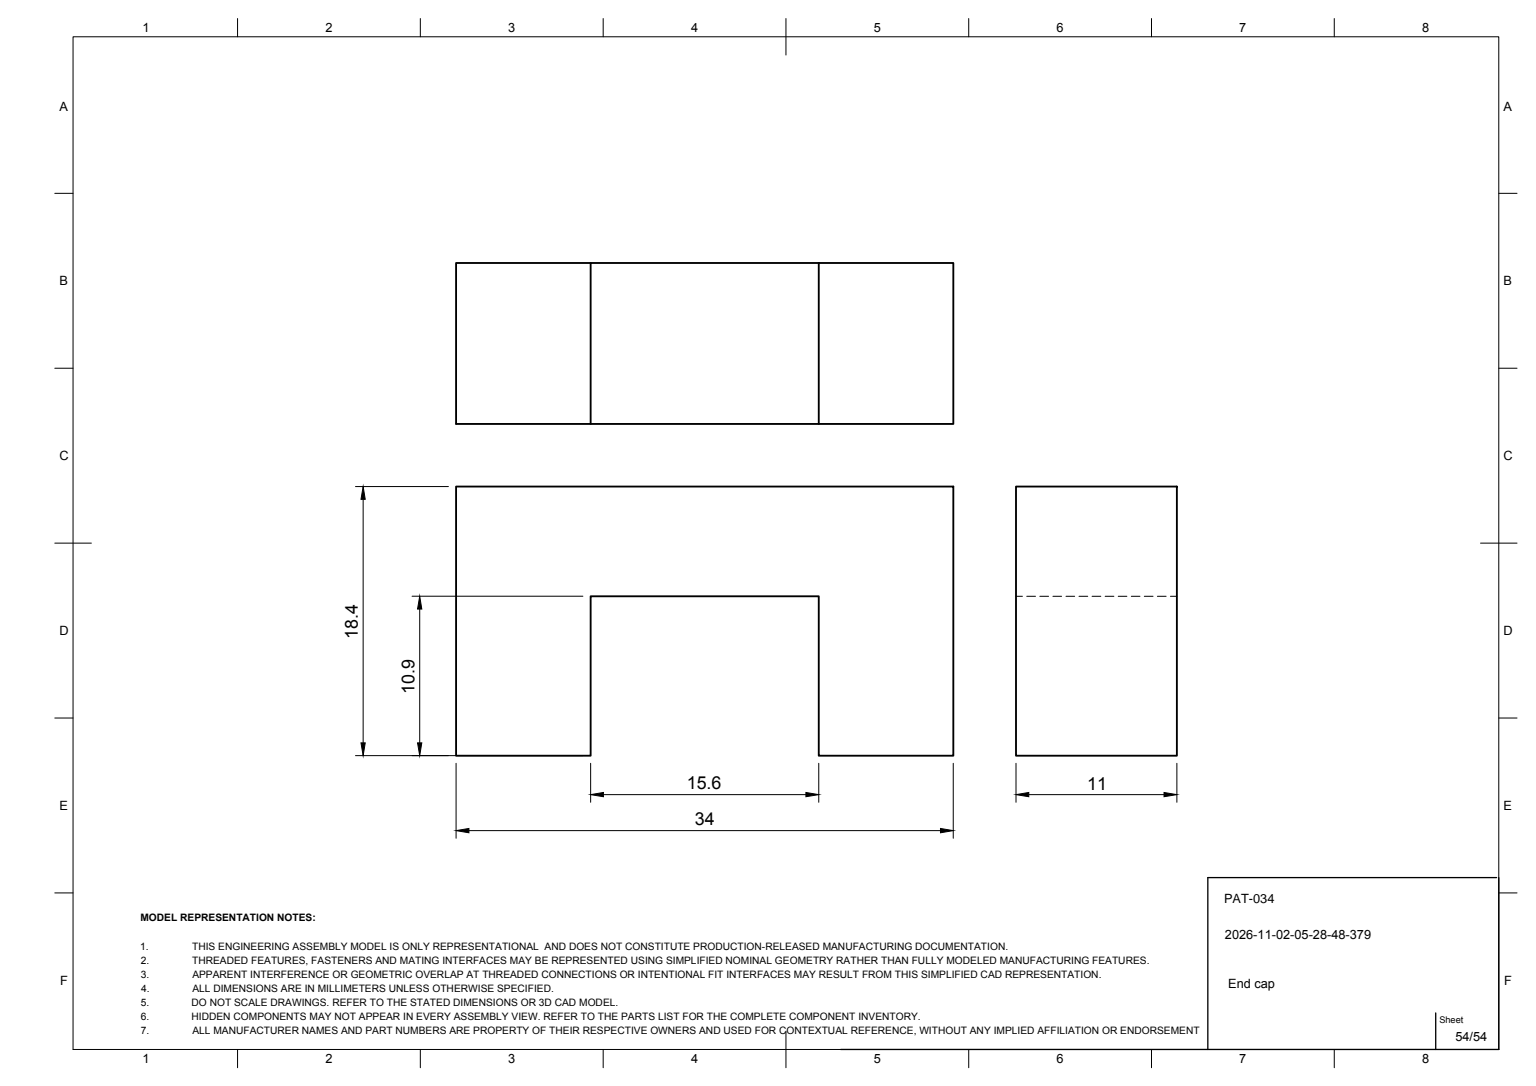
ISO-10303-21;
HEADER;
/* Generated by software containing ST-Developer
 * from STEP Tools, Inc. (www.steptools.com) 
 */

FILE_DESCRIPTION(
/* description */ ('Fatigue rig crank-slider'),
/* implementation_level */ '2;1');

FILE_NAME(
/* name */ 'End cap.step',
/* time_stamp */ '2026-10-28T03:24:50-07:00',
/* author */ (''),
/* organization */ (''),
/* preprocessor_version */ 'ST-DEVELOPER v20.2',
/* originating_system */ 'Autodesk Translation Framework v15.17.0.0',
/* authorisation */ '');

FILE_SCHEMA (('AUTOMOTIVE_DESIGN { 1 0 10303 214 3 1 1 }'));
ENDSEC;

DATA;
#10=MECHANICAL_DESIGN_GEOMETRIC_PRESENTATION_REPRESENTATION('',(#641),#16911);
#532=SHAPE_REPRESENTATION_RELATIONSHIP('SRR','None',#17177,#582);
#582=ADVANCED_BREP_SHAPE_REPRESENTATION('',(#698),#16906);
#641=STYLED_ITEM('',(#17501),#698);
#698=MANIFOLD_SOLID_BREP('Body1',#8934);
#1172=PLANE('',#10393);
#1173=PLANE('',#10394);
#1174=PLANE('',#10395);
#1175=PLANE('',#10396);
#1176=PLANE('',#10397);
#1177=PLANE('',#10398);
#1178=PLANE('',#10399);
#1179=PLANE('',#10400);
#1180=PLANE('',#10401);
#1181=PLANE('',#10402);
#1676=FACE_OUTER_BOUND('',#2391,.T.);
#1677=FACE_OUTER_BOUND('',#2392,.T.);
#1678=FACE_OUTER_BOUND('',#2393,.T.);
#1679=FACE_OUTER_BOUND('',#2394,.T.);
#1680=FACE_OUTER_BOUND('',#2395,.T.);
#1681=FACE_OUTER_BOUND('',#2396,.T.);
#1682=FACE_OUTER_BOUND('',#2397,.T.);
#1683=FACE_OUTER_BOUND('',#2398,.T.);
#1684=FACE_OUTER_BOUND('',#2399,.T.);
#1685=FACE_OUTER_BOUND('',#2400,.T.);
#2391=EDGE_LOOP('',(#7948,#7949,#7950,#7951));
#2392=EDGE_LOOP('',(#7952,#7953,#7954,#7955));
#2393=EDGE_LOOP('',(#7956,#7957,#7958,#7959));
#2394=EDGE_LOOP('',(#7960,#7961,#7962,#7963));
#2395=EDGE_LOOP('',(#7964,#7965,#7966,#7967));
#2396=EDGE_LOOP('',(#7968,#7969,#7970,#7971));
#2397=EDGE_LOOP('',(#7972,#7973,#7974,#7975));
#2398=EDGE_LOOP('',(#7976,#7977,#7978,#7979));
#2399=EDGE_LOOP('',(#7980,#7981,#7982,#7983,#7984,#7985,#7986,#7987));
#2400=EDGE_LOOP('',(#7988,#7989,#7990,#7991,#7992,#7993,#7994,#7995));
#3009=LINE('',#16448,#3655);
#3010=LINE('',#16450,#3656);
#3011=LINE('',#16452,#3657);
#3012=LINE('',#16453,#3658);
#3013=LINE('',#16456,#3659);
#3014=LINE('',#16458,#3660);
#3015=LINE('',#16459,#3661);
#3016=LINE('',#16462,#3662);
#3017=LINE('',#16464,#3663);
#3018=LINE('',#16465,#3664);
#3019=LINE('',#16468,#3665);
#3020=LINE('',#16470,#3666);
#3021=LINE('',#16471,#3667);
#3022=LINE('',#16474,#3668);
#3023=LINE('',#16476,#3669);
#3024=LINE('',#16477,#3670);
#3025=LINE('',#16480,#3671);
#3026=LINE('',#16482,#3672);
#3027=LINE('',#16483,#3673);
#3028=LINE('',#16486,#3674);
#3029=LINE('',#16488,#3675);
#3030=LINE('',#16489,#3676);
#3031=LINE('',#16491,#3677);
#3032=LINE('',#16492,#3678);
#3655=VECTOR('',#12917,1.);
#3656=VECTOR('',#12918,1.);
#3657=VECTOR('',#12919,1.);
#3658=VECTOR('',#12920,1.);
#3659=VECTOR('',#12923,1.);
#3660=VECTOR('',#12924,1.);
#3661=VECTOR('',#12925,1.);
#3662=VECTOR('',#12928,1.);
#3663=VECTOR('',#12929,1.);
#3664=VECTOR('',#12930,1.);
#3665=VECTOR('',#12933,1.);
#3666=VECTOR('',#12934,1.);
#3667=VECTOR('',#12935,1.);
#3668=VECTOR('',#12938,1.);
#3669=VECTOR('',#12939,1.);
#3670=VECTOR('',#12940,1.);
#3671=VECTOR('',#12943,1.);
#3672=VECTOR('',#12944,1.);
#3673=VECTOR('',#12945,1.);
#3674=VECTOR('',#12948,1.);
#3675=VECTOR('',#12949,1.);
#3676=VECTOR('',#12950,1.);
#3677=VECTOR('',#12953,1.);
#3678=VECTOR('',#12954,1.);
#4817=VERTEX_POINT('',#16446);
#4818=VERTEX_POINT('',#16447);
#4819=VERTEX_POINT('',#16449);
#4820=VERTEX_POINT('',#16451);
#4821=VERTEX_POINT('',#16455);
#4822=VERTEX_POINT('',#16457);
#4823=VERTEX_POINT('',#16461);
#4824=VERTEX_POINT('',#16463);
#4825=VERTEX_POINT('',#16467);
#4826=VERTEX_POINT('',#16469);
#4827=VERTEX_POINT('',#16473);
#4828=VERTEX_POINT('',#16475);
#4829=VERTEX_POINT('',#16479);
#4830=VERTEX_POINT('',#16481);
#4831=VERTEX_POINT('',#16485);
#4832=VERTEX_POINT('',#16487);
#5872=EDGE_CURVE('',#4817,#4818,#3009,.T.);
#5873=EDGE_CURVE('',#4817,#4819,#3010,.T.);
#5874=EDGE_CURVE('',#4820,#4819,#3011,.T.);
#5875=EDGE_CURVE('',#4818,#4820,#3012,.T.);
#5876=EDGE_CURVE('',#4818,#4821,#3013,.T.);
#5877=EDGE_CURVE('',#4822,#4820,#3014,.T.);
#5878=EDGE_CURVE('',#4821,#4822,#3015,.T.);
#5879=EDGE_CURVE('',#4821,#4823,#3016,.T.);
#5880=EDGE_CURVE('',#4824,#4822,#3017,.T.);
#5881=EDGE_CURVE('',#4823,#4824,#3018,.T.);
#5882=EDGE_CURVE('',#4823,#4825,#3019,.T.);
#5883=EDGE_CURVE('',#4826,#4824,#3020,.T.);
#5884=EDGE_CURVE('',#4825,#4826,#3021,.T.);
#5885=EDGE_CURVE('',#4825,#4827,#3022,.T.);
#5886=EDGE_CURVE('',#4828,#4826,#3023,.T.);
#5887=EDGE_CURVE('',#4827,#4828,#3024,.T.);
#5888=EDGE_CURVE('',#4827,#4829,#3025,.T.);
#5889=EDGE_CURVE('',#4830,#4828,#3026,.T.);
#5890=EDGE_CURVE('',#4829,#4830,#3027,.T.);
#5891=EDGE_CURVE('',#4829,#4831,#3028,.T.);
#5892=EDGE_CURVE('',#4832,#4830,#3029,.T.);
#5893=EDGE_CURVE('',#4831,#4832,#3030,.T.);
#5894=EDGE_CURVE('',#4831,#4817,#3031,.T.);
#5895=EDGE_CURVE('',#4819,#4832,#3032,.T.);
#7948=ORIENTED_EDGE('',*,*,#5872,.F.);
#7949=ORIENTED_EDGE('',*,*,#5873,.T.);
#7950=ORIENTED_EDGE('',*,*,#5874,.F.);
#7951=ORIENTED_EDGE('',*,*,#5875,.F.);
#7952=ORIENTED_EDGE('',*,*,#5876,.F.);
#7953=ORIENTED_EDGE('',*,*,#5875,.T.);
#7954=ORIENTED_EDGE('',*,*,#5877,.F.);
#7955=ORIENTED_EDGE('',*,*,#5878,.F.);
#7956=ORIENTED_EDGE('',*,*,#5879,.F.);
#7957=ORIENTED_EDGE('',*,*,#5878,.T.);
#7958=ORIENTED_EDGE('',*,*,#5880,.F.);
#7959=ORIENTED_EDGE('',*,*,#5881,.F.);
#7960=ORIENTED_EDGE('',*,*,#5882,.F.);
#7961=ORIENTED_EDGE('',*,*,#5881,.T.);
#7962=ORIENTED_EDGE('',*,*,#5883,.F.);
#7963=ORIENTED_EDGE('',*,*,#5884,.F.);
#7964=ORIENTED_EDGE('',*,*,#5885,.F.);
#7965=ORIENTED_EDGE('',*,*,#5884,.T.);
#7966=ORIENTED_EDGE('',*,*,#5886,.F.);
#7967=ORIENTED_EDGE('',*,*,#5887,.F.);
#7968=ORIENTED_EDGE('',*,*,#5888,.F.);
#7969=ORIENTED_EDGE('',*,*,#5887,.T.);
#7970=ORIENTED_EDGE('',*,*,#5889,.F.);
#7971=ORIENTED_EDGE('',*,*,#5890,.F.);
#7972=ORIENTED_EDGE('',*,*,#5891,.F.);
#7973=ORIENTED_EDGE('',*,*,#5890,.T.);
#7974=ORIENTED_EDGE('',*,*,#5892,.F.);
#7975=ORIENTED_EDGE('',*,*,#5893,.F.);
#7976=ORIENTED_EDGE('',*,*,#5894,.F.);
#7977=ORIENTED_EDGE('',*,*,#5893,.T.);
#7978=ORIENTED_EDGE('',*,*,#5895,.F.);
#7979=ORIENTED_EDGE('',*,*,#5873,.F.);
#7980=ORIENTED_EDGE('',*,*,#5894,.T.);
#7981=ORIENTED_EDGE('',*,*,#5872,.T.);
#7982=ORIENTED_EDGE('',*,*,#5876,.T.);
#7983=ORIENTED_EDGE('',*,*,#5879,.T.);
#7984=ORIENTED_EDGE('',*,*,#5882,.T.);
#7985=ORIENTED_EDGE('',*,*,#5885,.T.);
#7986=ORIENTED_EDGE('',*,*,#5888,.T.);
#7987=ORIENTED_EDGE('',*,*,#5891,.T.);
#7988=ORIENTED_EDGE('',*,*,#5895,.T.);
#7989=ORIENTED_EDGE('',*,*,#5892,.T.);
#7990=ORIENTED_EDGE('',*,*,#5889,.T.);
#7991=ORIENTED_EDGE('',*,*,#5886,.T.);
#7992=ORIENTED_EDGE('',*,*,#5883,.T.);
#7993=ORIENTED_EDGE('',*,*,#5880,.T.);
#7994=ORIENTED_EDGE('',*,*,#5877,.T.);
#7995=ORIENTED_EDGE('',*,*,#5874,.T.);
#8814=ADVANCED_FACE('',(#1676),#1172,.T.);
#8815=ADVANCED_FACE('',(#1677),#1173,.T.);
#8816=ADVANCED_FACE('',(#1678),#1174,.T.);
#8817=ADVANCED_FACE('',(#1679),#1175,.T.);
#8818=ADVANCED_FACE('',(#1680),#1176,.T.);
#8819=ADVANCED_FACE('',(#1681),#1177,.T.);
#8820=ADVANCED_FACE('',(#1682),#1178,.T.);
#8821=ADVANCED_FACE('',(#1683),#1179,.T.);
#8822=ADVANCED_FACE('',(#1684),#1180,.T.);
#8823=ADVANCED_FACE('',(#1685),#1181,.T.);
#8934=CLOSED_SHELL('',(#8814,#8815,#8816,#8817,#8818,#8819,#8820,#8821,
#8822,#8823));
#10392=AXIS2_PLACEMENT_3D('',#16444,#12913,#12914);
#10393=AXIS2_PLACEMENT_3D('',#16445,#12915,#12916);
#10394=AXIS2_PLACEMENT_3D('',#16454,#12921,#12922);
#10395=AXIS2_PLACEMENT_3D('',#16460,#12926,#12927);
#10396=AXIS2_PLACEMENT_3D('',#16466,#12931,#12932);
#10397=AXIS2_PLACEMENT_3D('',#16472,#12936,#12937);
#10398=AXIS2_PLACEMENT_3D('',#16478,#12941,#12942);
#10399=AXIS2_PLACEMENT_3D('',#16484,#12946,#12947);
#10400=AXIS2_PLACEMENT_3D('',#16490,#12951,#12952);
#10401=AXIS2_PLACEMENT_3D('',#16493,#12955,#12956);
#10402=AXIS2_PLACEMENT_3D('',#16494,#12957,#12958);
#12913=DIRECTION('axis',(0.,0.,1.));
#12914=DIRECTION('refdir',(1.,0.,0.));
#12915=DIRECTION('center_axis',(0.,0.,-1.));
#12916=DIRECTION('ref_axis',(0.,-1.,0.));
#12917=DIRECTION('',(0.,1.,0.));
#12918=DIRECTION('',(-1.,0.,0.));
#12919=DIRECTION('',(0.,-1.,0.));
#12920=DIRECTION('',(-1.,0.,0.));
#12921=DIRECTION('center_axis',(0.,1.,0.));
#12922=DIRECTION('ref_axis',(0.,0.,-1.));
#12923=DIRECTION('',(0.,0.,1.));
#12924=DIRECTION('',(0.,0.,-1.));
#12925=DIRECTION('',(-1.,0.,0.));
#12926=DIRECTION('center_axis',(0.,0.,-1.));
#12927=DIRECTION('ref_axis',(0.,-1.,0.));
#12928=DIRECTION('',(0.,1.,0.));
#12929=DIRECTION('',(0.,-1.,0.));
#12930=DIRECTION('',(-1.,0.,0.));
#12931=DIRECTION('center_axis',(0.,-1.,0.));
#12932=DIRECTION('ref_axis',(0.,0.,1.));
#12933=DIRECTION('',(0.,0.,-1.));
#12934=DIRECTION('',(0.,0.,1.));
#12935=DIRECTION('',(-1.,0.,0.));
#12936=DIRECTION('center_axis',(0.,0.,-1.));
#12937=DIRECTION('ref_axis',(0.,-1.,0.));
#12938=DIRECTION('',(0.,1.,0.));
#12939=DIRECTION('',(0.,-1.,0.));
#12940=DIRECTION('',(-1.,0.,0.));
#12941=DIRECTION('center_axis',(0.,1.,0.));
#12942=DIRECTION('ref_axis',(0.,0.,-1.));
#12943=DIRECTION('',(0.,0.,1.));
#12944=DIRECTION('',(0.,0.,-1.));
#12945=DIRECTION('',(-1.,0.,0.));
#12946=DIRECTION('center_axis',(0.,0.,1.));
#12947=DIRECTION('ref_axis',(0.,1.,0.));
#12948=DIRECTION('',(0.,-1.,0.));
#12949=DIRECTION('',(0.,1.,0.));
#12950=DIRECTION('',(-1.,0.,0.));
#12951=DIRECTION('center_axis',(0.,-1.,0.));
#12952=DIRECTION('ref_axis',(0.,0.,1.));
#12953=DIRECTION('',(0.,0.,-1.));
#12954=DIRECTION('',(0.,0.,1.));
#12955=DIRECTION('center_axis',(1.,0.,0.));
#12956=DIRECTION('ref_axis',(0.,0.,-1.));
#12957=DIRECTION('center_axis',(-1.,0.,0.));
#12958=DIRECTION('ref_axis',(0.,0.,1.));
#16444=CARTESIAN_POINT('',(0.,0.,0.));
#16445=CARTESIAN_POINT('Origin',(-1.97,-0.78,0.46));
#16446=CARTESIAN_POINT('',(-1.97,-1.7,0.46));
#16447=CARTESIAN_POINT('',(-1.97,-0.78,0.46));
#16448=CARTESIAN_POINT('',(-1.97,-1.7,0.46));
#16449=CARTESIAN_POINT('',(-3.07,-1.7,0.46));
#16450=CARTESIAN_POINT('',(-1.97,-1.7,0.46));
#16451=CARTESIAN_POINT('',(-3.07,-0.78,0.46));
#16452=CARTESIAN_POINT('',(-3.07,-1.7,0.46));
#16453=CARTESIAN_POINT('',(-1.97,-0.78,0.46));
#16454=CARTESIAN_POINT('Origin',(-1.97,-0.78,1.55));
#16455=CARTESIAN_POINT('',(-1.97,-0.78,1.55));
#16456=CARTESIAN_POINT('',(-1.97,-0.78,0.46));
#16457=CARTESIAN_POINT('',(-3.07,-0.78,1.55));
#16458=CARTESIAN_POINT('',(-3.07,-0.78,0.46));
#16459=CARTESIAN_POINT('',(-1.97,-0.78,1.55));
#16460=CARTESIAN_POINT('Origin',(-1.97,0.78,1.55));
#16461=CARTESIAN_POINT('',(-1.97,0.78,1.55));
#16462=CARTESIAN_POINT('',(-1.97,-0.78,1.55));
#16463=CARTESIAN_POINT('',(-3.07,0.78,1.55));
#16464=CARTESIAN_POINT('',(-3.07,-0.78,1.55));
#16465=CARTESIAN_POINT('',(-1.97,0.78,1.55));
#16466=CARTESIAN_POINT('Origin',(-1.97,0.78,0.46));
#16467=CARTESIAN_POINT('',(-1.97,0.78,0.46));
#16468=CARTESIAN_POINT('',(-1.97,0.78,1.55));
#16469=CARTESIAN_POINT('',(-3.07,0.78,0.46));
#16470=CARTESIAN_POINT('',(-3.07,0.78,1.55));
#16471=CARTESIAN_POINT('',(-1.97,0.78,0.46));
#16472=CARTESIAN_POINT('Origin',(-1.97,1.7,0.46));
#16473=CARTESIAN_POINT('',(-1.97,1.7,0.46));
#16474=CARTESIAN_POINT('',(-1.97,0.78,0.46));
#16475=CARTESIAN_POINT('',(-3.07,1.7,0.46));
#16476=CARTESIAN_POINT('',(-3.07,0.78,0.46));
#16477=CARTESIAN_POINT('',(-1.97,1.7,0.46));
#16478=CARTESIAN_POINT('Origin',(-1.97,1.7,2.3));
#16479=CARTESIAN_POINT('',(-1.97,1.7,2.3));
#16480=CARTESIAN_POINT('',(-1.97,1.7,0.46));
#16481=CARTESIAN_POINT('',(-3.07,1.7,2.3));
#16482=CARTESIAN_POINT('',(-3.07,1.7,0.46));
#16483=CARTESIAN_POINT('',(-1.97,1.7,2.3));
#16484=CARTESIAN_POINT('Origin',(-1.97,-1.7,2.3));
#16485=CARTESIAN_POINT('',(-1.97,-1.7,2.3));
#16486=CARTESIAN_POINT('',(-1.97,1.7,2.3));
#16487=CARTESIAN_POINT('',(-3.07,-1.7,2.3));
#16488=CARTESIAN_POINT('',(-3.07,1.7,2.3));
#16489=CARTESIAN_POINT('',(-1.97,-1.7,2.3));
#16490=CARTESIAN_POINT('Origin',(-1.97,-1.7,0.46));
#16491=CARTESIAN_POINT('',(-1.97,-1.7,2.3));
#16492=CARTESIAN_POINT('',(-3.07,-1.7,2.3));
#16493=CARTESIAN_POINT('Origin',(-1.97,0.,1.38));
#16494=CARTESIAN_POINT('Origin',(-3.07,0.,1.38));
#16847=UNCERTAINTY_MEASURE_WITH_UNIT(LENGTH_MEASURE(0.001),#16912,
'DISTANCE_ACCURACY_VALUE',
'Maximum model space distance between geometric entities at asserted c
onnectivities');
#16852=UNCERTAINTY_MEASURE_WITH_UNIT(LENGTH_MEASURE(0.001),#16912,
'DISTANCE_ACCURACY_VALUE',
'Maximum model space distance between geometric entities at asserted c
onnectivities');
#16906=(
GEOMETRIC_REPRESENTATION_CONTEXT(3)
GLOBAL_UNCERTAINTY_ASSIGNED_CONTEXT((#16847))
GLOBAL_UNIT_ASSIGNED_CONTEXT((#16912,#16914,#16915))
REPRESENTATION_CONTEXT('','3D')
);
#16911=(
GEOMETRIC_REPRESENTATION_CONTEXT(3)
GLOBAL_UNCERTAINTY_ASSIGNED_CONTEXT((#16852))
GLOBAL_UNIT_ASSIGNED_CONTEXT((#16912,#16914,#16915))
REPRESENTATION_CONTEXT('','3D')
);
#16912=(
LENGTH_UNIT()
NAMED_UNIT(*)
SI_UNIT(.CENTI.,.METRE.)
);
#16914=(
NAMED_UNIT(*)
PLANE_ANGLE_UNIT()
SI_UNIT($,.RADIAN.)
);
#16915=(
NAMED_UNIT(*)
SI_UNIT($,.STERADIAN.)
SOLID_ANGLE_UNIT()
);
#16969=SHAPE_DEFINITION_REPRESENTATION(#17041,#17177);
#17041=PRODUCT_DEFINITION_SHAPE('',$,#17236);
#17177=SHAPE_REPRESENTATION('',(#10392),#16906);
#17182=PRODUCT_DEFINITION_CONTEXT('part definition',#17358,'design');
#17236=PRODUCT_DEFINITION('End cap','End cap',#17294,#17182);
#17294=PRODUCT_DEFINITION_FORMATION('',$,#17413);
#17358=APPLICATION_CONTEXT(
'Core Data for Automotive Mechanical Design Process');
#17359=PRODUCT_CONTEXT('part definition',#17358,'mechanical');
#17413=PRODUCT('End cap','End cap','End cap',(#17359));
#17495=COLOUR_RGB('Off White',0.89,0.88,0.83);
#17496=FILL_AREA_STYLE_COLOUR('',#17495);
#17497=FILL_AREA_STYLE('',(#17496));
#17498=SURFACE_STYLE_FILL_AREA(#17497);
#17499=SURFACE_SIDE_STYLE('',(#17498));
#17500=SURFACE_STYLE_USAGE(.BOTH.,#17499);
#17501=PRESENTATION_STYLE_ASSIGNMENT((#17500));
ENDSEC;
END-ISO-10303-21;
